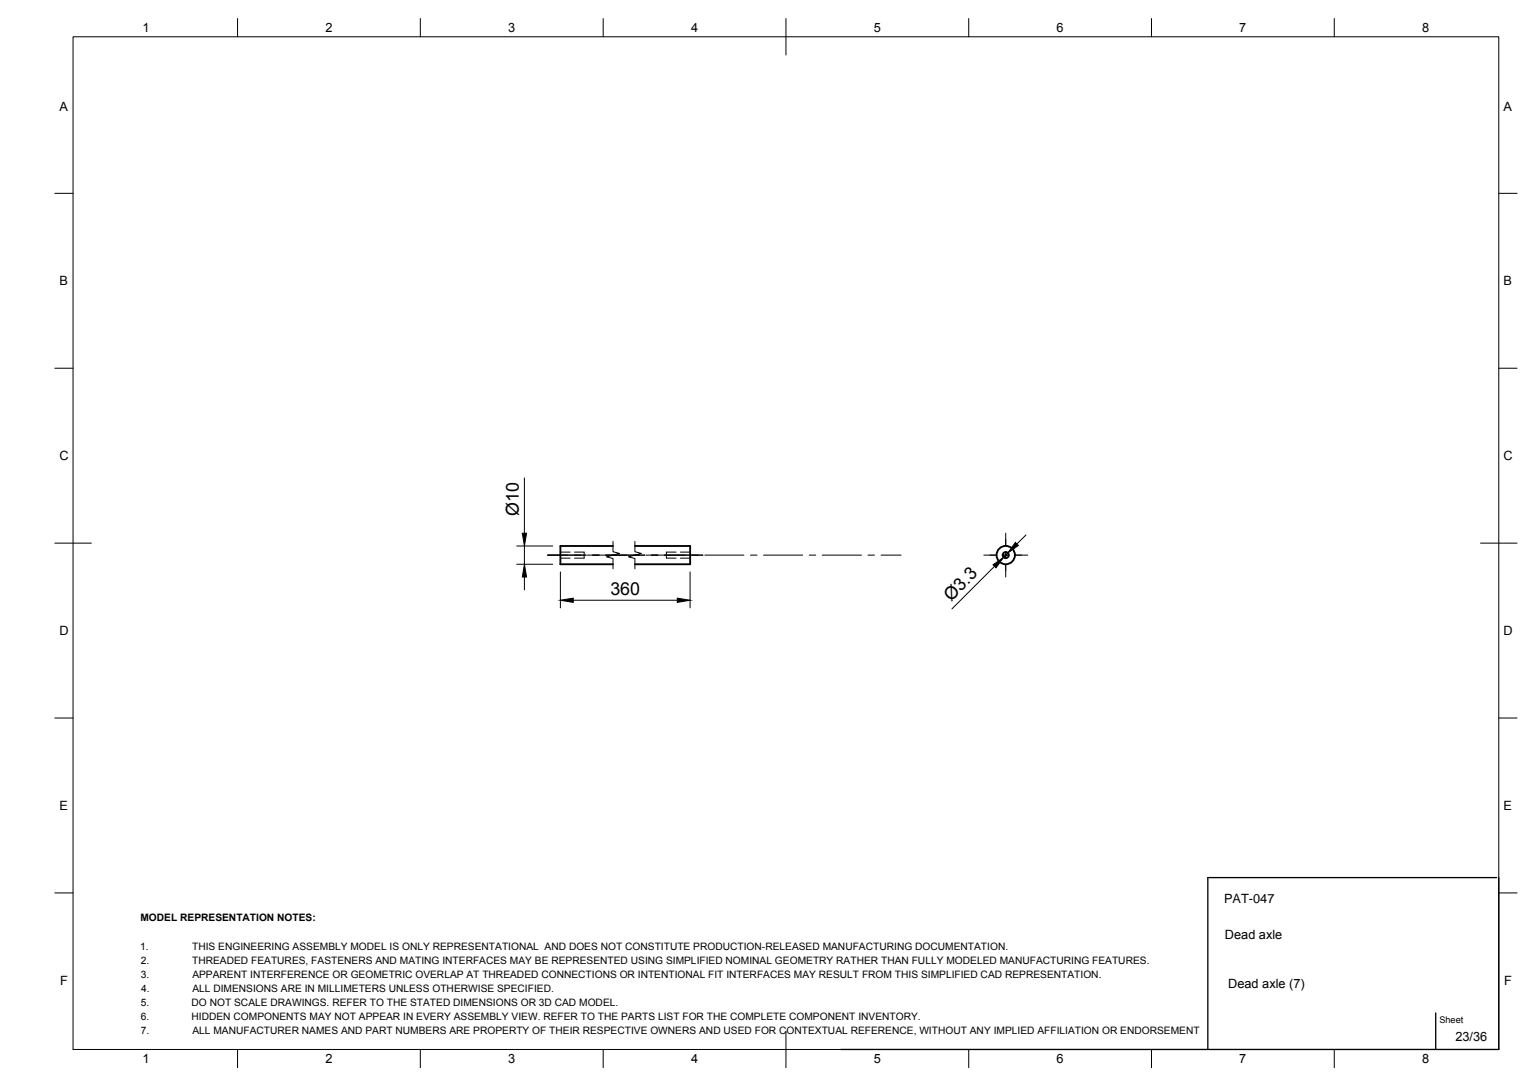
ISO-10303-21;
HEADER;
/* Generated by software containing ST-Developer
 * from STEP Tools, Inc. (www.steptools.com) 
 */

FILE_DESCRIPTION(
/* description */ ('Gravity roller conveyor section'),
/* implementation_level */ '2;1');

FILE_NAME(
/* name */ 'Dead axle.step',
/* time_stamp */ '2026-11-02T07:43:02-08:00',
/* author */ (''),
/* organization */ (''),
/* preprocessor_version */ 'ST-DEVELOPER v20.2',
/* originating_system */ 'Autodesk Translation Framework v15.17.0.0',
/* authorisation */ '');

FILE_SCHEMA (('AUTOMOTIVE_DESIGN { 1 0 10303 214 3 1 1 }'));
ENDSEC;

DATA;
#10=MECHANICAL_DESIGN_GEOMETRIC_PRESENTATION_REPRESENTATION('',(#548),#13821);
#480=SHAPE_REPRESENTATION_RELATIONSHIP('SRR','None',#14018,#514);
#514=ADVANCED_BREP_SHAPE_REPRESENTATION('',(#588),#13805);
#548=STYLED_ITEM('',(#14192),#588);
#588=MANIFOLD_SOLID_BREP('Body1',#7648);
#664=FACE_BOUND('',#1760,.T.);
#665=FACE_BOUND('',#1762,.T.);
#927=PLANE('',#8431);
#928=PLANE('',#8435);
#929=PLANE('',#8439);
#930=PLANE('',#8440);
#1280=FACE_OUTER_BOUND('',#1754,.T.);
#1281=FACE_OUTER_BOUND('',#1755,.T.);
#1282=FACE_OUTER_BOUND('',#1756,.T.);
#1283=FACE_OUTER_BOUND('',#1757,.T.);
#1284=FACE_OUTER_BOUND('',#1758,.T.);
#1285=FACE_OUTER_BOUND('',#1759,.T.);
#1286=FACE_OUTER_BOUND('',#1761,.T.);
#1754=EDGE_LOOP('',(#6546,#6547,#6548,#6549));
#1755=EDGE_LOOP('',(#6550));
#1756=EDGE_LOOP('',(#6551,#6552,#6553,#6554));
#1757=EDGE_LOOP('',(#6555));
#1758=EDGE_LOOP('',(#6556,#6557,#6558,#6559));
#1759=EDGE_LOOP('',(#6560));
#1760=EDGE_LOOP('',(#6561));
#1761=EDGE_LOOP('',(#6562));
#1762=EDGE_LOOP('',(#6563));
#2516=LINE('',#12661,#3234);
#2517=LINE('',#12668,#3235);
#2518=LINE('',#12675,#3236);
#3234=VECTOR('',#10159,0.165);
#3235=VECTOR('',#10168,0.165);
#3236=VECTOR('',#10177,0.5);
#3458=CIRCLE('',#8429,0.165);
#3459=CIRCLE('',#8430,0.165);
#3460=CIRCLE('',#8433,0.165);
#3461=CIRCLE('',#8434,0.165);
#3462=CIRCLE('',#8437,0.5);
#3463=CIRCLE('',#8438,0.5);
#4036=VERTEX_POINT('',#12658);
#4037=VERTEX_POINT('',#12660);
#4038=VERTEX_POINT('',#12665);
#4039=VERTEX_POINT('',#12667);
#4040=VERTEX_POINT('',#12672);
#4041=VERTEX_POINT('',#12674);
#4910=EDGE_CURVE('',#4036,#4036,#3458,.T.);
#4911=EDGE_CURVE('',#4036,#4037,#2516,.T.);
#4912=EDGE_CURVE('',#4037,#4037,#3459,.T.);
#4913=EDGE_CURVE('',#4038,#4038,#3460,.T.);
#4914=EDGE_CURVE('',#4038,#4039,#2517,.T.);
#4915=EDGE_CURVE('',#4039,#4039,#3461,.T.);
#4916=EDGE_CURVE('',#4040,#4040,#3462,.T.);
#4917=EDGE_CURVE('',#4040,#4041,#2518,.T.);
#4918=EDGE_CURVE('',#4041,#4041,#3463,.T.);
#6546=ORIENTED_EDGE('',*,*,#4910,.F.);
#6547=ORIENTED_EDGE('',*,*,#4911,.T.);
#6548=ORIENTED_EDGE('',*,*,#4912,.F.);
#6549=ORIENTED_EDGE('',*,*,#4911,.F.);
#6550=ORIENTED_EDGE('',*,*,#4910,.T.);
#6551=ORIENTED_EDGE('',*,*,#4913,.F.);
#6552=ORIENTED_EDGE('',*,*,#4914,.T.);
#6553=ORIENTED_EDGE('',*,*,#4915,.T.);
#6554=ORIENTED_EDGE('',*,*,#4914,.F.);
#6555=ORIENTED_EDGE('',*,*,#4915,.F.);
#6556=ORIENTED_EDGE('',*,*,#4916,.F.);
#6557=ORIENTED_EDGE('',*,*,#4917,.T.);
#6558=ORIENTED_EDGE('',*,*,#4918,.T.);
#6559=ORIENTED_EDGE('',*,*,#4917,.F.);
#6560=ORIENTED_EDGE('',*,*,#4916,.T.);
#6561=ORIENTED_EDGE('',*,*,#4912,.T.);
#6562=ORIENTED_EDGE('',*,*,#4918,.F.);
#6563=ORIENTED_EDGE('',*,*,#4913,.T.);
#7170=CYLINDRICAL_SURFACE('',#8428,0.165);
#7171=CYLINDRICAL_SURFACE('',#8432,0.165);
#7172=CYLINDRICAL_SURFACE('',#8436,0.5);
#7481=ADVANCED_FACE('',(#1280),#7170,.F.);
#7482=ADVANCED_FACE('',(#1281),#927,.T.);
#7483=ADVANCED_FACE('',(#1282),#7171,.F.);
#7484=ADVANCED_FACE('',(#1283),#928,.F.);
#7485=ADVANCED_FACE('',(#1284),#7172,.T.);
#7486=ADVANCED_FACE('',(#1285,#664),#929,.T.);
#7487=ADVANCED_FACE('',(#1286,#665),#930,.F.);
#7648=CLOSED_SHELL('',(#7481,#7482,#7483,#7484,#7485,#7486,#7487));
#8427=AXIS2_PLACEMENT_3D('',#12656,#10153,#10154);
#8428=AXIS2_PLACEMENT_3D('',#12657,#10155,#10156);
#8429=AXIS2_PLACEMENT_3D('',#12659,#10157,#10158);
#8430=AXIS2_PLACEMENT_3D('',#12662,#10160,#10161);
#8431=AXIS2_PLACEMENT_3D('',#12663,#10162,#10163);
#8432=AXIS2_PLACEMENT_3D('',#12664,#10164,#10165);
#8433=AXIS2_PLACEMENT_3D('',#12666,#10166,#10167);
#8434=AXIS2_PLACEMENT_3D('',#12669,#10169,#10170);
#8435=AXIS2_PLACEMENT_3D('',#12670,#10171,#10172);
#8436=AXIS2_PLACEMENT_3D('',#12671,#10173,#10174);
#8437=AXIS2_PLACEMENT_3D('',#12673,#10175,#10176);
#8438=AXIS2_PLACEMENT_3D('',#12676,#10178,#10179);
#8439=AXIS2_PLACEMENT_3D('',#12677,#10180,#10181);
#8440=AXIS2_PLACEMENT_3D('',#12678,#10182,#10183);
#10153=DIRECTION('axis',(0.,0.,1.));
#10154=DIRECTION('refdir',(1.,0.,0.));
#10155=DIRECTION('center_axis',(0.,1.,0.));
#10156=DIRECTION('ref_axis',(1.,0.,0.));
#10157=DIRECTION('center_axis',(0.,1.,0.));
#10158=DIRECTION('ref_axis',(1.,0.,0.));
#10159=DIRECTION('',(0.,1.,0.));
#10160=DIRECTION('center_axis',(0.,-1.,0.));
#10161=DIRECTION('ref_axis',(1.,0.,0.));
#10162=DIRECTION('center_axis',(0.,1.,0.));
#10163=DIRECTION('ref_axis',(1.,0.,0.));
#10164=DIRECTION('center_axis',(0.,1.,0.));
#10165=DIRECTION('ref_axis',(1.,0.,0.));
#10166=DIRECTION('center_axis',(0.,1.,0.));
#10167=DIRECTION('ref_axis',(1.,0.,0.));
#10168=DIRECTION('',(0.,1.,0.));
#10169=DIRECTION('center_axis',(0.,1.,0.));
#10170=DIRECTION('ref_axis',(1.,0.,0.));
#10171=DIRECTION('center_axis',(0.,1.,0.));
#10172=DIRECTION('ref_axis',(1.,0.,0.));
#10173=DIRECTION('center_axis',(0.,1.,0.));
#10174=DIRECTION('ref_axis',(1.,0.,0.));
#10175=DIRECTION('center_axis',(0.,1.,0.));
#10176=DIRECTION('ref_axis',(1.,0.,0.));
#10177=DIRECTION('',(0.,-1.,0.));
#10178=DIRECTION('center_axis',(0.,1.,0.));
#10179=DIRECTION('ref_axis',(1.,0.,0.));
#10180=DIRECTION('center_axis',(0.,1.,0.));
#10181=DIRECTION('ref_axis',(1.,0.,0.));
#10182=DIRECTION('center_axis',(0.,1.,0.));
#10183=DIRECTION('ref_axis',(1.,0.,0.));
#12656=CARTESIAN_POINT('',(0.,0.,0.));
#12657=CARTESIAN_POINT('Origin',(3.,31.7,8.));
#12658=CARTESIAN_POINT('',(2.835,31.7,8.));
#12659=CARTESIAN_POINT('Origin',(3.,31.7,8.));
#12660=CARTESIAN_POINT('',(2.835,33.,8.));
#12661=CARTESIAN_POINT('',(2.835,31.7,8.));
#12662=CARTESIAN_POINT('Origin',(3.,33.,8.));
#12663=CARTESIAN_POINT('Origin',(3.,31.7,8.));
#12664=CARTESIAN_POINT('Origin',(3.,-3.1,8.));
#12665=CARTESIAN_POINT('',(2.835,-3.,8.));
#12666=CARTESIAN_POINT('Origin',(3.,-3.,8.));
#12667=CARTESIAN_POINT('',(2.835,-1.7,8.));
#12668=CARTESIAN_POINT('',(2.835,-3.1,8.));
#12669=CARTESIAN_POINT('Origin',(3.,-1.7,8.));
#12670=CARTESIAN_POINT('Origin',(3.,-1.7,8.));
#12671=CARTESIAN_POINT('Origin',(3.,-3.,8.));
#12672=CARTESIAN_POINT('',(2.5,33.,8.));
#12673=CARTESIAN_POINT('Origin',(3.,33.,8.));
#12674=CARTESIAN_POINT('',(2.5,-3.,8.));
#12675=CARTESIAN_POINT('',(2.5,-3.,8.));
#12676=CARTESIAN_POINT('Origin',(3.,-3.,8.));
#12677=CARTESIAN_POINT('Origin',(3.,33.,8.));
#12678=CARTESIAN_POINT('Origin',(3.,-3.,8.));
#13766=UNCERTAINTY_MEASURE_WITH_UNIT(LENGTH_MEASURE(0.001),#13822,
'DISTANCE_ACCURACY_VALUE',
'Maximum model space distance between geometric entities at asserted c
onnectivities');
#13782=UNCERTAINTY_MEASURE_WITH_UNIT(LENGTH_MEASURE(0.001),#13822,
'DISTANCE_ACCURACY_VALUE',
'Maximum model space distance between geometric entities at asserted c
onnectivities');
#13805=(
GEOMETRIC_REPRESENTATION_CONTEXT(3)
GLOBAL_UNCERTAINTY_ASSIGNED_CONTEXT((#13766))
GLOBAL_UNIT_ASSIGNED_CONTEXT((#13822,#13824,#13825))
REPRESENTATION_CONTEXT('','3D')
);
#13821=(
GEOMETRIC_REPRESENTATION_CONTEXT(3)
GLOBAL_UNCERTAINTY_ASSIGNED_CONTEXT((#13782))
GLOBAL_UNIT_ASSIGNED_CONTEXT((#13822,#13824,#13825))
REPRESENTATION_CONTEXT('','3D')
);
#13822=(
LENGTH_UNIT()
NAMED_UNIT(*)
SI_UNIT(.CENTI.,.METRE.)
);
#13824=(
NAMED_UNIT(*)
PLANE_ANGLE_UNIT()
SI_UNIT($,.RADIAN.)
);
#13825=(
NAMED_UNIT(*)
SI_UNIT($,.STERADIAN.)
SOLID_ANGLE_UNIT()
);
#13848=SHAPE_DEFINITION_REPRESENTATION(#13886,#14018);
#13886=PRODUCT_DEFINITION_SHAPE('',$,#14057);
#14018=SHAPE_REPRESENTATION('',(#8427),#13805);
#14034=PRODUCT_DEFINITION_CONTEXT('part definition',#14150,'design');
#14057=PRODUCT_DEFINITION('Dead axle','Dead axle',#14095,#14034);
#14095=PRODUCT_DEFINITION_FORMATION('',$,#14174);
#14150=APPLICATION_CONTEXT(
'Core Data for Automotive Mechanical Design Process');
#14151=PRODUCT_CONTEXT('part definition',#14150,'mechanical');
#14174=PRODUCT('Dead axle','Dead axle','Dead axle',(#14151));
#14192=PRESENTATION_STYLE_ASSIGNMENT((#14197));
#14197=SURFACE_STYLE_USAGE(.BOTH.,#14202);
#14202=SURFACE_SIDE_STYLE('',(#14207));
#14207=SURFACE_STYLE_FILL_AREA(#14212);
#14212=FILL_AREA_STYLE('CAD Library Painted - Engineering blue',(#14217));
#14217=FILL_AREA_STYLE_COLOUR('CAD Library Painted - Engineering blue',
#14222);
#14222=COLOUR_RGB('CAD Library Painted - Engineering blue',0.12156862745098,
0.356862745098039,0.6);
ENDSEC;
END-ISO-10303-21;
